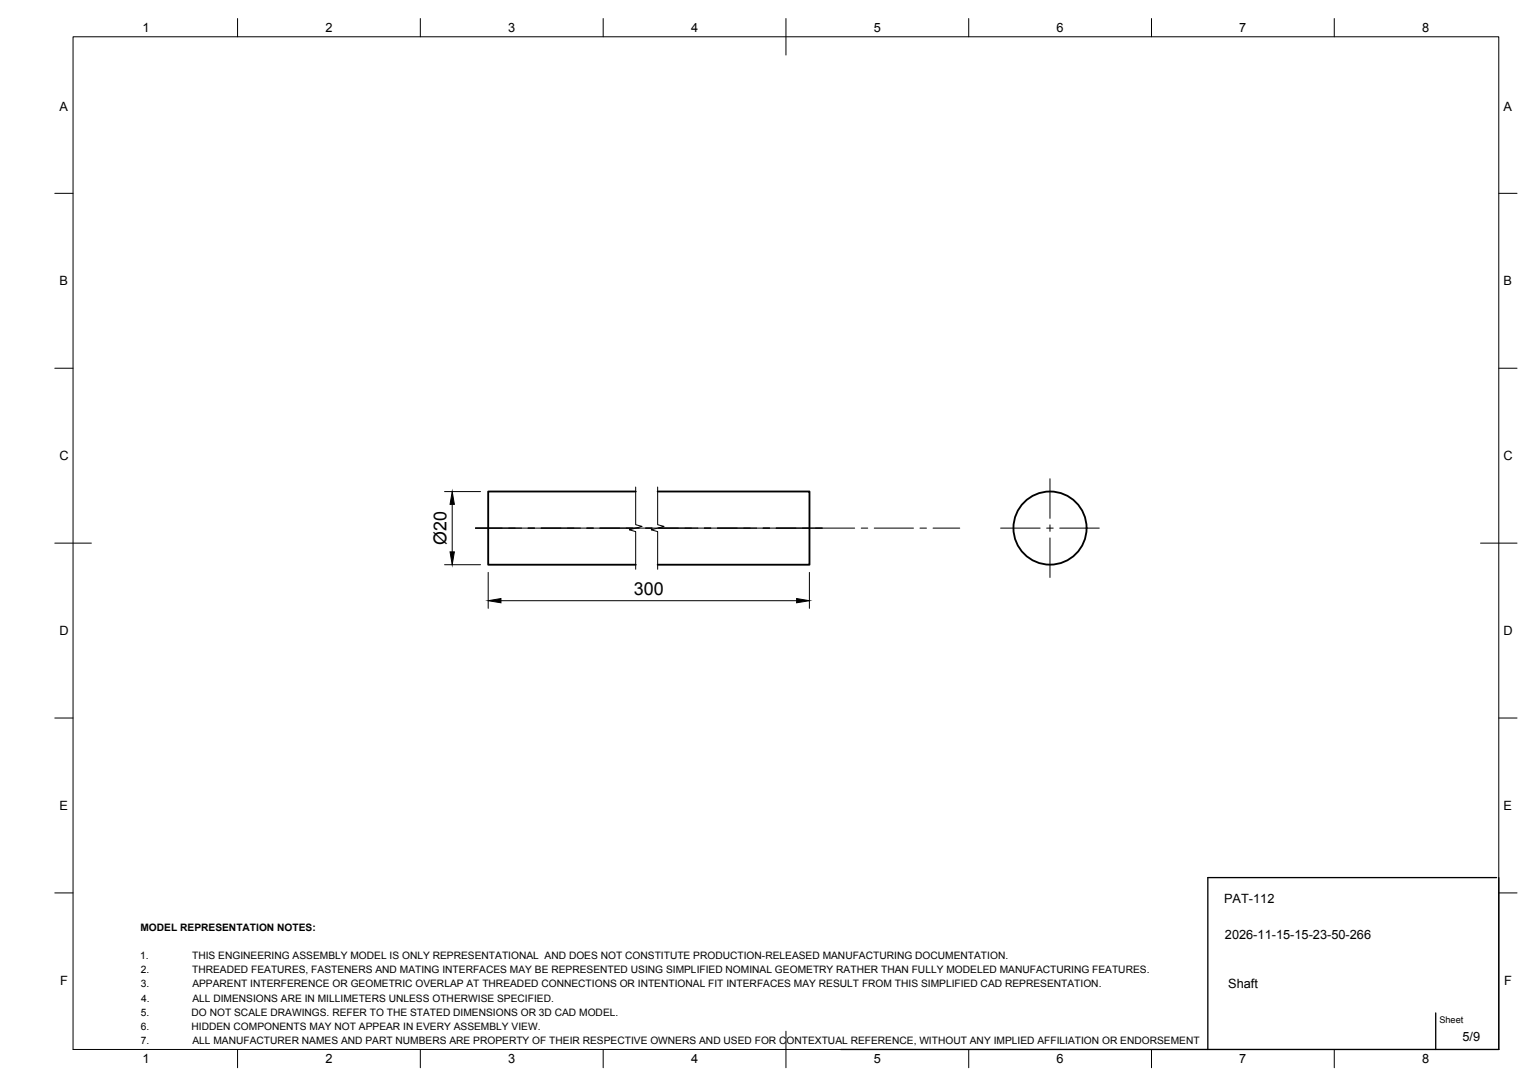
ISO-10303-21;
HEADER;
/* Generated by software containing ST-Developer
 * from STEP Tools, Inc. (www.steptools.com) 
 */

FILE_DESCRIPTION(
/* description */ ('PAT-112'),
/* implementation_level */ '2;1');

FILE_NAME(
/* name */ 'Shaft.step',
/* time_stamp */ '2026-11-15T15:25:42-08:00',
/* author */ (''),
/* organization */ (''),
/* preprocessor_version */ 'ST-DEVELOPER v20.2',
/* originating_system */ 'Autodesk Translation Framework v15.17.0.0',
/* authorisation */ '');

FILE_SCHEMA (('AUTOMOTIVE_DESIGN { 1 0 10303 214 3 1 1 }'));
ENDSEC;

DATA;
#10=MECHANICAL_DESIGN_GEOMETRIC_PRESENTATION_REPRESENTATION('',(#112),#2277);
#97=SHAPE_REPRESENTATION_RELATIONSHIP('SRR','None',#2326,#104);
#104=ADVANCED_BREP_SHAPE_REPRESENTATION('',(#119),#2276);
#112=STYLED_ITEM('',(#2367),#119);
#119=MANIFOLD_SOLID_BREP('Body1',#1265);
#195=PLANE('',#1479);
#196=PLANE('',#1483);
#271=FACE_OUTER_BOUND('',#374,.T.);
#272=FACE_OUTER_BOUND('',#375,.T.);
#273=FACE_OUTER_BOUND('',#376,.T.);
#374=EDGE_LOOP('',(#1154));
#375=EDGE_LOOP('',(#1155,#1156,#1157,#1158));
#376=EDGE_LOOP('',(#1159));
#471=LINE('',#2240,#566);
#566=VECTOR('',#1872,1.);
#617=CIRCLE('',#1480,1.);
#618=CIRCLE('',#1482,1.);
#717=VERTEX_POINT('',#2235);
#718=VERTEX_POINT('',#2238);
#863=EDGE_CURVE('',#717,#717,#617,.T.);
#864=EDGE_CURVE('',#718,#718,#618,.T.);
#865=EDGE_CURVE('',#718,#717,#471,.T.);
#1154=ORIENTED_EDGE('',*,*,#863,.T.);
#1155=ORIENTED_EDGE('',*,*,#864,.F.);
#1156=ORIENTED_EDGE('',*,*,#865,.T.);
#1157=ORIENTED_EDGE('',*,*,#863,.F.);
#1158=ORIENTED_EDGE('',*,*,#865,.F.);
#1159=ORIENTED_EDGE('',*,*,#864,.T.);
#1179=CYLINDRICAL_SURFACE('',#1481,1.);
#1254=ADVANCED_FACE('',(#271),#195,.F.);
#1255=ADVANCED_FACE('',(#272),#1179,.T.);
#1256=ADVANCED_FACE('',(#273),#196,.T.);
#1265=CLOSED_SHELL('',(#1254,#1255,#1256));
#1478=AXIS2_PLACEMENT_3D('',#2233,#1862,#1863);
#1479=AXIS2_PLACEMENT_3D('',#2234,#1864,#1865);
#1480=AXIS2_PLACEMENT_3D('',#2236,#1866,#1867);
#1481=AXIS2_PLACEMENT_3D('',#2237,#1868,#1869);
#1482=AXIS2_PLACEMENT_3D('',#2239,#1870,#1871);
#1483=AXIS2_PLACEMENT_3D('',#2241,#1873,#1874);
#1862=DIRECTION('axis',(0.,0.,1.));
#1863=DIRECTION('refdir',(1.,0.,0.));
#1864=DIRECTION('center_axis',(0.,1.,0.));
#1865=DIRECTION('ref_axis',(1.,0.,0.));
#1866=DIRECTION('center_axis',(0.,-1.,0.));
#1867=DIRECTION('ref_axis',(1.,0.,0.));
#1868=DIRECTION('center_axis',(0.,1.,0.));
#1869=DIRECTION('ref_axis',(1.,0.,0.));
#1870=DIRECTION('center_axis',(0.,1.,0.));
#1871=DIRECTION('ref_axis',(1.,0.,0.));
#1872=DIRECTION('',(0.,-1.,0.));
#1873=DIRECTION('center_axis',(0.,1.,0.));
#1874=DIRECTION('ref_axis',(1.,0.,0.));
#2233=CARTESIAN_POINT('',(0.,0.,0.));
#2234=CARTESIAN_POINT('Origin',(0.,-5.,4.53));
#2235=CARTESIAN_POINT('',(-1.,-5.,4.53));
#2236=CARTESIAN_POINT('Origin',(0.,-5.,4.53));
#2237=CARTESIAN_POINT('Origin',(0.,0.,4.53));
#2238=CARTESIAN_POINT('',(-1.,25.,4.53));
#2239=CARTESIAN_POINT('Origin',(0.,25.,4.53));
#2240=CARTESIAN_POINT('',(-1.,0.,4.53));
#2241=CARTESIAN_POINT('Origin',(0.,25.,4.53));
#2266=UNCERTAINTY_MEASURE_WITH_UNIT(LENGTH_MEASURE(0.001),#2278,
'DISTANCE_ACCURACY_VALUE',
'Maximum model space distance between geometric entities at asserted c
onnectivities');
#2267=UNCERTAINTY_MEASURE_WITH_UNIT(LENGTH_MEASURE(0.001),#2278,
'DISTANCE_ACCURACY_VALUE',
'Maximum model space distance between geometric entities at asserted c
onnectivities');
#2276=(
GEOMETRIC_REPRESENTATION_CONTEXT(3)
GLOBAL_UNCERTAINTY_ASSIGNED_CONTEXT((#2266))
GLOBAL_UNIT_ASSIGNED_CONTEXT((#2278,#2280,#2281))
REPRESENTATION_CONTEXT('','3D')
);
#2277=(
GEOMETRIC_REPRESENTATION_CONTEXT(3)
GLOBAL_UNCERTAINTY_ASSIGNED_CONTEXT((#2267))
GLOBAL_UNIT_ASSIGNED_CONTEXT((#2278,#2280,#2281))
REPRESENTATION_CONTEXT('','3D')
);
#2278=(
LENGTH_UNIT()
NAMED_UNIT(*)
SI_UNIT(.CENTI.,.METRE.)
);
#2280=(
NAMED_UNIT(*)
PLANE_ANGLE_UNIT()
SI_UNIT($,.RADIAN.)
);
#2281=(
NAMED_UNIT(*)
SI_UNIT($,.STERADIAN.)
SOLID_ANGLE_UNIT()
);
#2290=SHAPE_DEFINITION_REPRESENTATION(#2301,#2326);
#2301=PRODUCT_DEFINITION_SHAPE('',$,#2336);
#2326=SHAPE_REPRESENTATION('',(#1478),#2276);
#2327=PRODUCT_DEFINITION_CONTEXT('part definition',#2356,'design');
#2336=PRODUCT_DEFINITION('2026-11-15-15-23-50-266','Shaft',#2345,#2327);
#2345=PRODUCT_DEFINITION_FORMATION('',$,#2366);
#2356=APPLICATION_CONTEXT(
'Core Data for Automotive Mechanical Design Process');
#2357=PRODUCT_CONTEXT('part definition',#2356,'mechanical');
#2366=PRODUCT('2026-11-15-15-23-50-266','Shaft',$,(#2357));
#2367=PRESENTATION_STYLE_ASSIGNMENT((#2372));
#2372=SURFACE_STYLE_USAGE(.BOTH.,#2377);
#2377=SURFACE_SIDE_STYLE('',(#2382));
#2382=SURFACE_STYLE_FILL_AREA(#2387);
#2387=FILL_AREA_STYLE('Steel - Satin',(#2392));
#2392=FILL_AREA_STYLE_COLOUR('Steel - Satin',#2397);
#2397=COLOUR_RGB('Steel - Satin',0.627450980392157,0.627450980392157,0.627450980392157);
ENDSEC;
END-ISO-10303-21;
